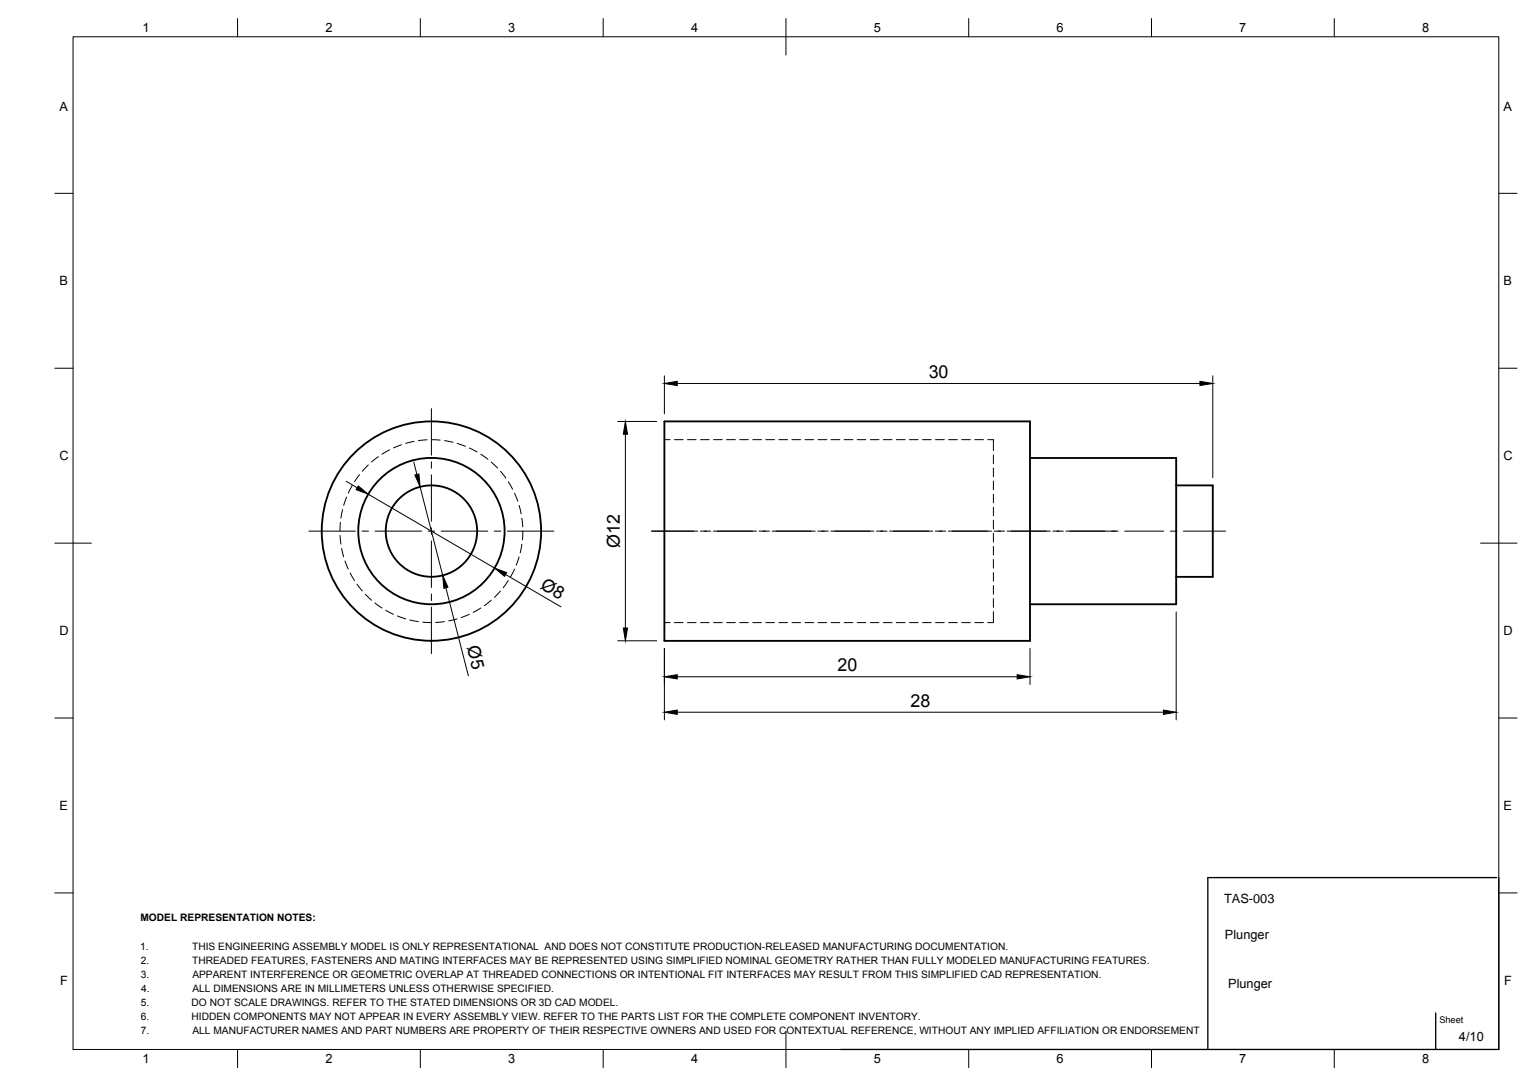
ISO-10303-21;
HEADER;
/* Generated by software containing ST-Developer
 * from STEP Tools, Inc. (www.steptools.com) 
 */

FILE_DESCRIPTION(
/* description */ ('STEP AP214'),
/* implementation_level */ '2;1');

FILE_NAME(
/* name */ 'Plunger.step',
/* time_stamp */ '2026-11-04T19:43:37-08:00',
/* author */ (''),
/* organization */ (''),
/* preprocessor_version */ 'ST-DEVELOPER v20.2',
/* originating_system */ 'Autodesk Translation Framework v15.17.0.0',
/* authorisation */ '');

FILE_SCHEMA (('AUTOMOTIVE_DESIGN { 1 0 10303 214 3 1 1 }'));
ENDSEC;

DATA;
#10=MECHANICAL_DESIGN_GEOMETRIC_PRESENTATION_REPRESENTATION('',(#116),#7627);
#98=SHAPE_REPRESENTATION_RELATIONSHIP('SRR','None',#7666,#107);
#107=ADVANCED_BREP_SHAPE_REPRESENTATION('',(#137),#7619);
#116=STYLED_ITEM('',(#7720),#137);
#137=MANIFOLD_SOLID_BREP('Body1',#2414);
#164=FACE_BOUND('',#494,.T.);
#165=FACE_BOUND('',#497,.T.);
#166=FACE_BOUND('',#499,.T.);
#200=PLANE('',#2585);
#201=PLANE('',#2586);
#202=PLANE('',#2587);
#203=PLANE('',#2588);
#204=PLANE('',#2589);
#262=CYLINDRICAL_SURFACE('',#2573,5.);
#263=CYLINDRICAL_SURFACE('',#2576,6.);
#264=CYLINDRICAL_SURFACE('',#2579,2.5);
#265=CYLINDRICAL_SURFACE('',#2582,4.);
#328=FACE_OUTER_BOUND('',#489,.T.);
#329=FACE_OUTER_BOUND('',#490,.T.);
#330=FACE_OUTER_BOUND('',#491,.T.);
#331=FACE_OUTER_BOUND('',#492,.T.);
#332=FACE_OUTER_BOUND('',#493,.T.);
#333=FACE_OUTER_BOUND('',#495,.T.);
#334=FACE_OUTER_BOUND('',#496,.T.);
#335=FACE_OUTER_BOUND('',#498,.T.);
#336=FACE_OUTER_BOUND('',#500,.T.);
#489=EDGE_LOOP('',(#1711,#1712,#1713,#1714));
#490=EDGE_LOOP('',(#1715,#1716,#1717,#1718));
#491=EDGE_LOOP('',(#1719,#1720,#1721,#1722));
#492=EDGE_LOOP('',(#1723,#1724,#1725,#1726));
#493=EDGE_LOOP('',(#1727));
#494=EDGE_LOOP('',(#1728));
#495=EDGE_LOOP('',(#1729));
#496=EDGE_LOOP('',(#1730));
#497=EDGE_LOOP('',(#1731));
#498=EDGE_LOOP('',(#1732));
#499=EDGE_LOOP('',(#1733));
#500=EDGE_LOOP('',(#1734));
#663=CIRCLE('',#2574,5.);
#664=CIRCLE('',#2575,5.);
#665=CIRCLE('',#2577,6.);
#666=CIRCLE('',#2578,6.);
#667=CIRCLE('',#2580,2.5);
#668=CIRCLE('',#2581,2.5);
#669=CIRCLE('',#2583,4.);
#670=CIRCLE('',#2584,4.);
#832=LINE('',#3782,#988);
#833=LINE('',#3788,#989);
#834=LINE('',#3794,#990);
#835=LINE('',#3800,#991);
#988=VECTOR('',#2975,5.);
#989=VECTOR('',#2982,6.);
#990=VECTOR('',#2989,2.5);
#991=VECTOR('',#2996,4.);
#1145=VERTEX_POINT('',#3779);
#1146=VERTEX_POINT('',#3781);
#1147=VERTEX_POINT('',#3785);
#1148=VERTEX_POINT('',#3787);
#1149=VERTEX_POINT('',#3791);
#1150=VERTEX_POINT('',#3793);
#1151=VERTEX_POINT('',#3797);
#1152=VERTEX_POINT('',#3799);
#1350=EDGE_CURVE('',#1145,#1145,#663,.T.);
#1351=EDGE_CURVE('',#1145,#1146,#832,.T.);
#1352=EDGE_CURVE('',#1146,#1146,#664,.T.);
#1353=EDGE_CURVE('',#1147,#1147,#665,.T.);
#1354=EDGE_CURVE('',#1147,#1148,#833,.T.);
#1355=EDGE_CURVE('',#1148,#1148,#666,.T.);
#1356=EDGE_CURVE('',#1149,#1149,#667,.T.);
#1357=EDGE_CURVE('',#1149,#1150,#834,.T.);
#1358=EDGE_CURVE('',#1150,#1150,#668,.T.);
#1359=EDGE_CURVE('',#1151,#1151,#669,.T.);
#1360=EDGE_CURVE('',#1151,#1152,#835,.T.);
#1361=EDGE_CURVE('',#1152,#1152,#670,.T.);
#1711=ORIENTED_EDGE('',*,*,#1350,.F.);
#1712=ORIENTED_EDGE('',*,*,#1351,.T.);
#1713=ORIENTED_EDGE('',*,*,#1352,.T.);
#1714=ORIENTED_EDGE('',*,*,#1351,.F.);
#1715=ORIENTED_EDGE('',*,*,#1353,.F.);
#1716=ORIENTED_EDGE('',*,*,#1354,.T.);
#1717=ORIENTED_EDGE('',*,*,#1355,.T.);
#1718=ORIENTED_EDGE('',*,*,#1354,.F.);
#1719=ORIENTED_EDGE('',*,*,#1356,.F.);
#1720=ORIENTED_EDGE('',*,*,#1357,.T.);
#1721=ORIENTED_EDGE('',*,*,#1358,.T.);
#1722=ORIENTED_EDGE('',*,*,#1357,.F.);
#1723=ORIENTED_EDGE('',*,*,#1359,.F.);
#1724=ORIENTED_EDGE('',*,*,#1360,.T.);
#1725=ORIENTED_EDGE('',*,*,#1361,.F.);
#1726=ORIENTED_EDGE('',*,*,#1360,.F.);
#1727=ORIENTED_EDGE('',*,*,#1359,.T.);
#1728=ORIENTED_EDGE('',*,*,#1358,.F.);
#1729=ORIENTED_EDGE('',*,*,#1356,.T.);
#1730=ORIENTED_EDGE('',*,*,#1355,.F.);
#1731=ORIENTED_EDGE('',*,*,#1361,.T.);
#1732=ORIENTED_EDGE('',*,*,#1353,.T.);
#1733=ORIENTED_EDGE('',*,*,#1352,.F.);
#1734=ORIENTED_EDGE('',*,*,#1350,.T.);
#2279=ADVANCED_FACE('',(#328),#262,.F.);
#2280=ADVANCED_FACE('',(#329),#263,.T.);
#2281=ADVANCED_FACE('',(#330),#264,.T.);
#2282=ADVANCED_FACE('',(#331),#265,.T.);
#2283=ADVANCED_FACE('',(#332,#164),#200,.T.);
#2284=ADVANCED_FACE('',(#333),#201,.F.);
#2285=ADVANCED_FACE('',(#334,#165),#202,.F.);
#2286=ADVANCED_FACE('',(#335,#166),#203,.T.);
#2287=ADVANCED_FACE('',(#336),#204,.T.);
#2414=CLOSED_SHELL('',(#2279,#2280,#2281,#2282,#2283,#2284,#2285,#2286,
#2287));
#2572=AXIS2_PLACEMENT_3D('',#3777,#2969,#2970);
#2573=AXIS2_PLACEMENT_3D('',#3778,#2971,#2972);
#2574=AXIS2_PLACEMENT_3D('',#3780,#2973,#2974);
#2575=AXIS2_PLACEMENT_3D('',#3783,#2976,#2977);
#2576=AXIS2_PLACEMENT_3D('',#3784,#2978,#2979);
#2577=AXIS2_PLACEMENT_3D('',#3786,#2980,#2981);
#2578=AXIS2_PLACEMENT_3D('',#3789,#2983,#2984);
#2579=AXIS2_PLACEMENT_3D('',#3790,#2985,#2986);
#2580=AXIS2_PLACEMENT_3D('',#3792,#2987,#2988);
#2581=AXIS2_PLACEMENT_3D('',#3795,#2990,#2991);
#2582=AXIS2_PLACEMENT_3D('',#3796,#2992,#2993);
#2583=AXIS2_PLACEMENT_3D('',#3798,#2994,#2995);
#2584=AXIS2_PLACEMENT_3D('',#3801,#2997,#2998);
#2585=AXIS2_PLACEMENT_3D('',#3802,#2999,#3000);
#2586=AXIS2_PLACEMENT_3D('',#3803,#3001,#3002);
#2587=AXIS2_PLACEMENT_3D('',#3804,#3003,#3004);
#2588=AXIS2_PLACEMENT_3D('',#3805,#3005,#3006);
#2589=AXIS2_PLACEMENT_3D('',#3806,#3007,#3008);
#2969=DIRECTION('axis',(0.,0.,1.));
#2970=DIRECTION('refdir',(1.,0.,0.));
#2971=DIRECTION('center_axis',(0.,1.,0.));
#2972=DIRECTION('ref_axis',(0.,0.,1.));
#2973=DIRECTION('center_axis',(0.,1.,0.));
#2974=DIRECTION('ref_axis',(0.,0.,1.));
#2975=DIRECTION('',(0.,1.,0.));
#2976=DIRECTION('center_axis',(0.,1.,0.));
#2977=DIRECTION('ref_axis',(0.,0.,1.));
#2978=DIRECTION('center_axis',(0.,1.,0.));
#2979=DIRECTION('ref_axis',(0.,0.,1.));
#2980=DIRECTION('center_axis',(0.,1.,0.));
#2981=DIRECTION('ref_axis',(0.,0.,1.));
#2982=DIRECTION('',(0.,-1.,0.));
#2983=DIRECTION('center_axis',(0.,1.,0.));
#2984=DIRECTION('ref_axis',(0.,0.,1.));
#2985=DIRECTION('center_axis',(0.,-1.,0.));
#2986=DIRECTION('ref_axis',(0.,0.,-1.));
#2987=DIRECTION('center_axis',(0.,-1.,0.));
#2988=DIRECTION('ref_axis',(0.,0.,-1.));
#2989=DIRECTION('',(0.,1.,0.));
#2990=DIRECTION('center_axis',(0.,-1.,0.));
#2991=DIRECTION('ref_axis',(0.,0.,-1.));
#2992=DIRECTION('center_axis',(0.,-1.,0.));
#2993=DIRECTION('ref_axis',(0.,0.,-1.));
#2994=DIRECTION('center_axis',(0.,-1.,0.));
#2995=DIRECTION('ref_axis',(0.,0.,-1.));
#2996=DIRECTION('',(0.,1.,0.));
#2997=DIRECTION('center_axis',(0.,1.,0.));
#2998=DIRECTION('ref_axis',(0.,0.,1.));
#2999=DIRECTION('center_axis',(0.,-1.,0.));
#3000=DIRECTION('ref_axis',(0.,0.,-1.));
#3001=DIRECTION('center_axis',(0.,1.,0.));
#3002=DIRECTION('ref_axis',(0.,0.,1.));
#3003=DIRECTION('center_axis',(0.,1.,0.));
#3004=DIRECTION('ref_axis',(0.,0.,1.));
#3005=DIRECTION('center_axis',(0.,1.,0.));
#3006=DIRECTION('ref_axis',(0.,0.,1.));
#3007=DIRECTION('center_axis',(0.,1.,0.));
#3008=DIRECTION('ref_axis',(0.,0.,1.));
#3777=CARTESIAN_POINT('',(0.,0.,0.));
#3778=CARTESIAN_POINT('Origin',(0.,15.,0.));
#3779=CARTESIAN_POINT('',(-6.12323399573677E-16,15.,-5.));
#3780=CARTESIAN_POINT('Origin',(0.,15.,0.));
#3781=CARTESIAN_POINT('',(-6.12323399573677E-16,33.,-5.));
#3782=CARTESIAN_POINT('',(-6.12323399573677E-16,15.,-5.));
#3783=CARTESIAN_POINT('Origin',(0.,33.,0.));
#3784=CARTESIAN_POINT('Origin',(0.,13.,0.));
#3785=CARTESIAN_POINT('',(-7.34788079488412E-16,33.,-6.));
#3786=CARTESIAN_POINT('Origin',(0.,33.,0.));
#3787=CARTESIAN_POINT('',(-7.34788079488412E-16,13.,-6.));
#3788=CARTESIAN_POINT('',(-7.34788079488412E-16,13.,-6.));
#3789=CARTESIAN_POINT('Origin',(0.,13.,0.));
#3790=CARTESIAN_POINT('Origin',(0.,5.,0.));
#3791=CARTESIAN_POINT('',(-3.06161699786838E-16,3.,2.5));
#3792=CARTESIAN_POINT('Origin',(0.,3.,0.));
#3793=CARTESIAN_POINT('',(-3.06161699786838E-16,5.,2.5));
#3794=CARTESIAN_POINT('',(-3.06161699786838E-16,5.,2.5));
#3795=CARTESIAN_POINT('Origin',(0.,5.,0.));
#3796=CARTESIAN_POINT('Origin',(0.,33.,0.));
#3797=CARTESIAN_POINT('',(-4.89858719658941E-16,5.,4.));
#3798=CARTESIAN_POINT('Origin',(0.,5.,0.));
#3799=CARTESIAN_POINT('',(-4.89858719658941E-16,13.,4.));
#3800=CARTESIAN_POINT('',(-4.89858719658941E-16,33.,4.));
#3801=CARTESIAN_POINT('Origin',(0.,13.,0.));
#3802=CARTESIAN_POINT('Origin',(0.,5.,0.));
#3803=CARTESIAN_POINT('Origin',(0.,3.,0.));
#3804=CARTESIAN_POINT('Origin',(0.,13.,0.));
#3805=CARTESIAN_POINT('Origin',(0.,33.,0.));
#3806=CARTESIAN_POINT('Origin',(0.,15.,0.));
#7608=UNCERTAINTY_MEASURE_WITH_UNIT(LENGTH_MEASURE(0.01),#7628,
'DISTANCE_ACCURACY_VALUE',
'Maximum model space distance between geometric entities at asserted c
onnectivities');
#7616=UNCERTAINTY_MEASURE_WITH_UNIT(LENGTH_MEASURE(0.01),#7628,
'DISTANCE_ACCURACY_VALUE',
'Maximum model space distance between geometric entities at asserted c
onnectivities');
#7619=(
GEOMETRIC_REPRESENTATION_CONTEXT(3)
GLOBAL_UNCERTAINTY_ASSIGNED_CONTEXT((#7608))
GLOBAL_UNIT_ASSIGNED_CONTEXT((#7628,#7630,#7631))
REPRESENTATION_CONTEXT('','3D')
);
#7627=(
GEOMETRIC_REPRESENTATION_CONTEXT(3)
GLOBAL_UNCERTAINTY_ASSIGNED_CONTEXT((#7616))
GLOBAL_UNIT_ASSIGNED_CONTEXT((#7628,#7630,#7631))
REPRESENTATION_CONTEXT('','3D')
);
#7628=(
LENGTH_UNIT()
NAMED_UNIT(*)
SI_UNIT(.MILLI.,.METRE.)
);
#7630=(
NAMED_UNIT(*)
PLANE_ANGLE_UNIT()
SI_UNIT($,.RADIAN.)
);
#7631=(
NAMED_UNIT(*)
SI_UNIT($,.STERADIAN.)
SOLID_ANGLE_UNIT()
);
#7634=SHAPE_DEFINITION_REPRESENTATION(#7644,#7666);
#7644=PRODUCT_DEFINITION_SHAPE('',$,#7677);
#7666=SHAPE_REPRESENTATION('',(#2572),#7619);
#7674=PRODUCT_DEFINITION_CONTEXT('part definition',#7706,'design');
#7677=PRODUCT_DEFINITION('Plunger','Plunger',#7687,#7674);
#7687=PRODUCT_DEFINITION_FORMATION('',$,#7710);
#7706=APPLICATION_CONTEXT(
'Core Data for Automotive Mechanical Design Process');
#7707=PRODUCT_CONTEXT('part definition',#7706,'mechanical');
#7710=PRODUCT('Plunger','Plunger',$,(#7707));
#7720=PRESENTATION_STYLE_ASSIGNMENT((#7726));
#7726=SURFACE_STYLE_USAGE(.BOTH.,#7732);
#7732=SURFACE_SIDE_STYLE('',(#7738));
#7738=SURFACE_STYLE_FILL_AREA(#7744);
#7744=FILL_AREA_STYLE('Opaque(227,224,212)',(#7750));
#7750=FILL_AREA_STYLE_COLOUR('Opaque(227,224,212)',#7756);
#7756=COLOUR_RGB('Opaque(227,224,212)',0.890196078431372,0.87843137254902,
0.831372549019608);
ENDSEC;
END-ISO-10303-21;
